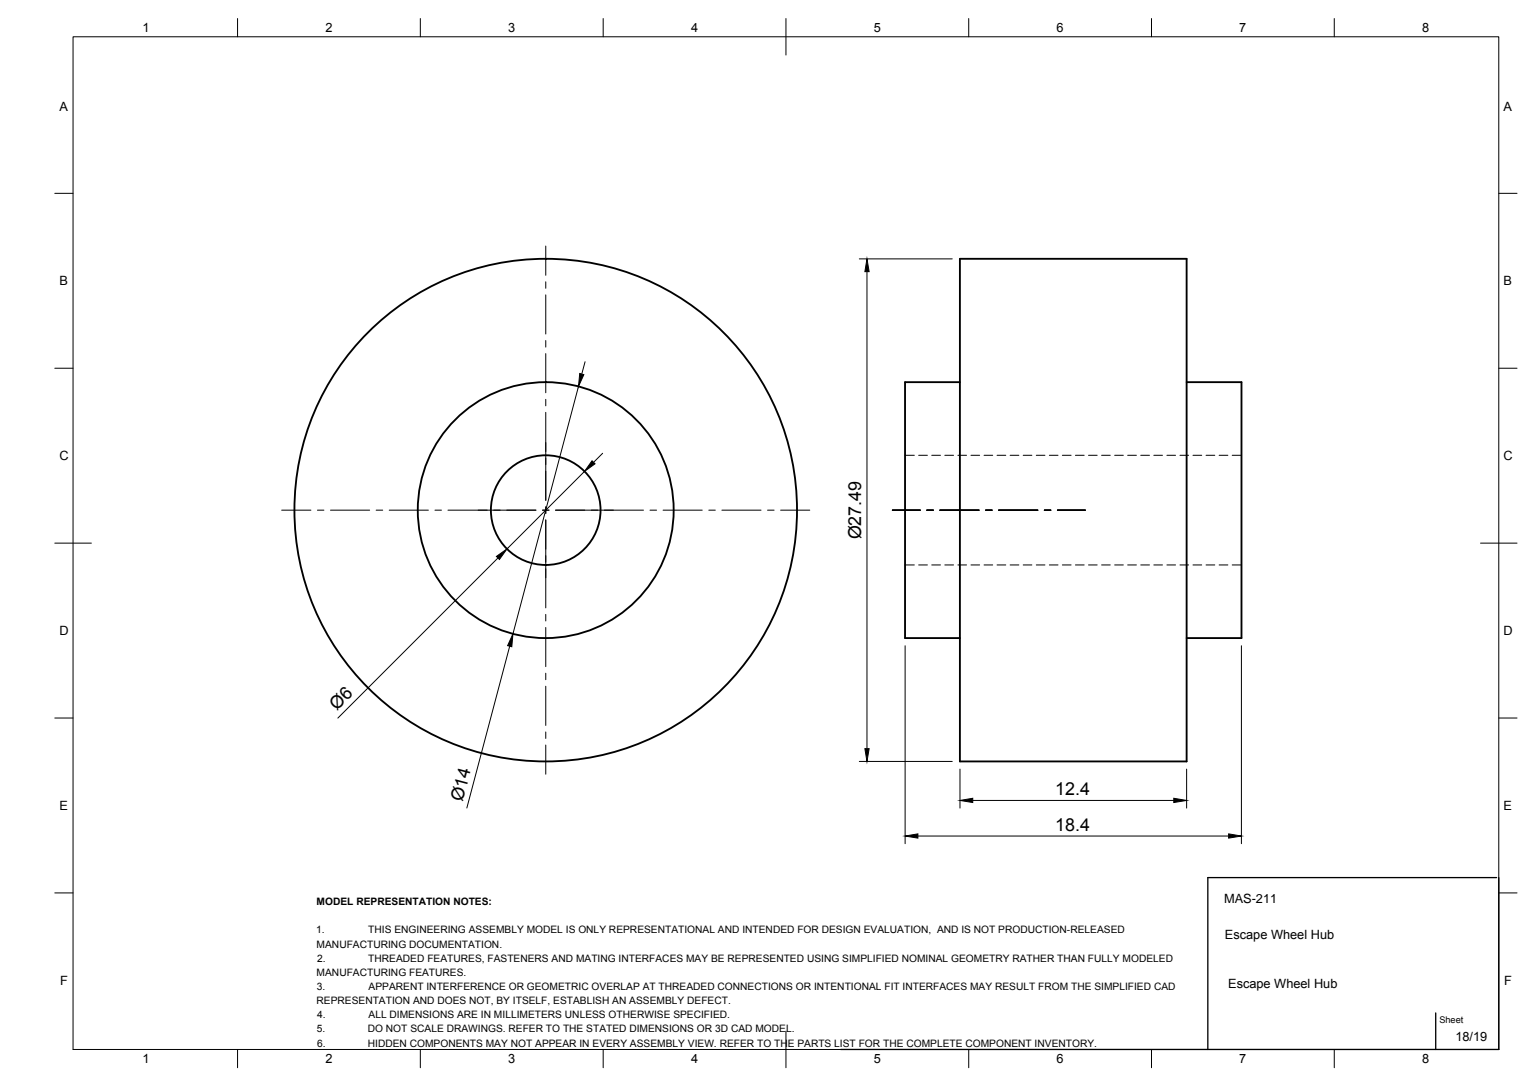
ISO-10303-21;
HEADER;
FILE_DESCRIPTION(
 (''),
 '2;1');
FILE_NAME ( 'Escape Wheel Hub.step', '2026-10-05T20:07:59+06:00', ( '' ), ( '' ), 'STEP AP214', 'Unspecified', '' );
FILE_SCHEMA (('AUTOMOTIVE_DESIGN { 1 0 10303 214 3 1 1 }'));
ENDSEC;
DATA;
#10=MECHANICAL_DESIGN_GEOMETRIC_PRESENTATION_REPRESENTATION('',(#336),#196741);
#336=STYLED_ITEM('',(#196765),#355) ;
#355=MANIFOLD_SOLID_BREP('Escape Wheel Hub',#8732) ;
#416=PLANE('',#9088) ;
#417=PLANE('',#9091) ;
#418=PLANE('',#9096) ;
#419=PLANE('',#9098) ;
#594=FACE_BOUND('',#1612,.T.) ;
#595=FACE_BOUND('',#1614,.T.) ;
#596=FACE_BOUND('',#1617,.T.) ;
#597=FACE_BOUND('',#1619,.T.) ;
#737=CIRCLE('',#9086,7.) ;
#738=CIRCLE('',#9087,7.) ;
#739=CIRCLE('',#9089,7.) ;
#740=CIRCLE('',#9090,3.00000000000006) ;
#741=CIRCLE('',#9092,3.00000000000006) ;
#742=CIRCLE('',#9094,13.7469842874597) ;
#743=CIRCLE('',#9095,13.7469842874597) ;
#744=CIRCLE('',#9097,7.) ;
#1097=FACE_OUTER_BOUND('',#1610,.T.) ;
#1098=FACE_OUTER_BOUND('',#1611,.T.) ;
#1099=FACE_OUTER_BOUND('',#1613,.T.) ;
#1100=FACE_OUTER_BOUND('',#1615,.T.) ;
#1101=FACE_OUTER_BOUND('',#1616,.T.) ;
#1102=FACE_OUTER_BOUND('',#1618,.T.) ;
#1103=FACE_OUTER_BOUND('',#1620,.T.) ;
#1104=FACE_OUTER_BOUND('',#1621,.T.) ;
#1610=EDGE_LOOP('',(#6758,#6759,#6760,#6761)) ;
#1611=EDGE_LOOP('',(#6762)) ;
#1612=EDGE_LOOP('',(#6763)) ;
#1613=EDGE_LOOP('',(#6764)) ;
#1614=EDGE_LOOP('',(#6765)) ;
#1615=EDGE_LOOP('',(#6766,#6767,#6768,#6769)) ;
#1616=EDGE_LOOP('',(#6770)) ;
#1617=EDGE_LOOP('',(#6771)) ;
#1618=EDGE_LOOP('',(#6772)) ;
#1619=EDGE_LOOP('',(#6773)) ;
#1620=EDGE_LOOP('',(#6774,#6775,#6776,#6777)) ;
#1621=EDGE_LOOP('',(#6778,#6779,#6780,#6781)) ;
#2079=LINE('',#194829,#2782) ;
#2080=LINE('',#194843,#2783) ;
#2081=LINE('',#194850,#2784) ;
#2082=LINE('',#194852,#2785) ;
#2782=VECTOR('',#10353,7.00000000000021) ;
#2783=VECTOR('',#10370,13.7469842874597) ;
#2784=VECTOR('',#10381,7.00000000000021) ;
#2785=VECTOR('',#10384,3.00000000000005) ;
#3838=VERTEX_POINT('',#194826) ;
#3839=VERTEX_POINT('',#194828) ;
#3840=VERTEX_POINT('',#194832) ;
#3841=VERTEX_POINT('',#194834) ;
#3842=VERTEX_POINT('',#194837) ;
#3843=VERTEX_POINT('',#194840) ;
#3844=VERTEX_POINT('',#194842) ;
#3845=VERTEX_POINT('',#194846) ;
#4887=EDGE_CURVE('',#3838,#3838,#737,.T.) ;
#4888=EDGE_CURVE('',#3838,#3839,#2079,.T.) ;
#4889=EDGE_CURVE('',#3839,#3839,#738,.T.) ;
#4890=EDGE_CURVE('',#3840,#3840,#739,.T.) ;
#4891=EDGE_CURVE('',#3841,#3841,#740,.T.) ;
#4892=EDGE_CURVE('',#3842,#3842,#741,.T.) ;
#4893=EDGE_CURVE('',#3843,#3843,#742,.T.) ;
#4894=EDGE_CURVE('',#3843,#3844,#2080,.T.) ;
#4895=EDGE_CURVE('',#3844,#3844,#743,.T.) ;
#4896=EDGE_CURVE('',#3845,#3845,#744,.T.) ;
#4897=EDGE_CURVE('',#3840,#3845,#2081,.T.) ;
#4898=EDGE_CURVE('',#3842,#3841,#2082,.T.) ;
#6758=ORIENTED_EDGE('',*,*,#4887,.T.) ;
#6759=ORIENTED_EDGE('',*,*,#4888,.T.) ;
#6760=ORIENTED_EDGE('',*,*,#4889,.F.) ;
#6761=ORIENTED_EDGE('',*,*,#4888,.F.) ;
#6762=ORIENTED_EDGE('',*,*,#4890,.F.) ;
#6763=ORIENTED_EDGE('',*,*,#4891,.F.) ;
#6764=ORIENTED_EDGE('',*,*,#4889,.T.) ;
#6765=ORIENTED_EDGE('',*,*,#4892,.T.) ;
#6766=ORIENTED_EDGE('',*,*,#4893,.T.) ;
#6767=ORIENTED_EDGE('',*,*,#4894,.T.) ;
#6768=ORIENTED_EDGE('',*,*,#4895,.F.) ;
#6769=ORIENTED_EDGE('',*,*,#4894,.F.) ;
#6770=ORIENTED_EDGE('',*,*,#4893,.F.) ;
#6771=ORIENTED_EDGE('',*,*,#4896,.T.) ;
#6772=ORIENTED_EDGE('',*,*,#4895,.T.) ;
#6773=ORIENTED_EDGE('',*,*,#4887,.F.) ;
#6774=ORIENTED_EDGE('',*,*,#4890,.T.) ;
#6775=ORIENTED_EDGE('',*,*,#4897,.T.) ;
#6776=ORIENTED_EDGE('',*,*,#4896,.F.) ;
#6777=ORIENTED_EDGE('',*,*,#4897,.F.) ;
#6778=ORIENTED_EDGE('',*,*,#4892,.F.) ;
#6779=ORIENTED_EDGE('',*,*,#4898,.T.) ;
#6780=ORIENTED_EDGE('',*,*,#4891,.T.) ;
#6781=ORIENTED_EDGE('',*,*,#4898,.F.) ;
#8205=CYLINDRICAL_SURFACE('',#9085,7.00000000000021) ;
#8206=CYLINDRICAL_SURFACE('',#9093,13.7469842874597) ;
#8207=CYLINDRICAL_SURFACE('',#9099,7.00000000000021) ;
#8208=CYLINDRICAL_SURFACE('',#9100,3.00000000000005) ;
#8480=ADVANCED_FACE('',(#1097),#8205,.T.) ;
#8481=ADVANCED_FACE('',(#1098,#594),#416,.T.) ;
#8482=ADVANCED_FACE('',(#1099,#595),#417,.T.) ;
#8483=ADVANCED_FACE('',(#1100),#8206,.T.) ;
#8484=ADVANCED_FACE('',(#1101,#596),#418,.T.) ;
#8485=ADVANCED_FACE('',(#1102,#597),#419,.T.) ;
#8486=ADVANCED_FACE('',(#1103),#8207,.T.) ;
#8487=ADVANCED_FACE('',(#1104),#8208,.F.) ;
#8732=CLOSED_SHELL('',(#8480,#8481,#8482,#8483,#8484,#8485,#8486,#8487)) ;
#9085=AXIS2_PLACEMENT_3D('',#194825,#10349,#10350) ;
#9086=AXIS2_PLACEMENT_3D('',#194827,#10351,#10352) ;
#9087=AXIS2_PLACEMENT_3D('',#194830,#10354,#10355) ;
#9088=AXIS2_PLACEMENT_3D('',#194831,#10356,#10357) ;
#9089=AXIS2_PLACEMENT_3D('',#194833,#10358,#10359) ;
#9090=AXIS2_PLACEMENT_3D('',#194835,#10360,#10361) ;
#9091=AXIS2_PLACEMENT_3D('',#194836,#10362,#10363) ;
#9092=AXIS2_PLACEMENT_3D('',#194838,#10364,#10365) ;
#9093=AXIS2_PLACEMENT_3D('',#194839,#10366,#10367) ;
#9094=AXIS2_PLACEMENT_3D('',#194841,#10368,#10369) ;
#9095=AXIS2_PLACEMENT_3D('',#194844,#10371,#10372) ;
#9096=AXIS2_PLACEMENT_3D('',#194845,#10373,#10374) ;
#9097=AXIS2_PLACEMENT_3D('',#194847,#10375,#10376) ;
#9098=AXIS2_PLACEMENT_3D('',#194848,#10377,#10378) ;
#9099=AXIS2_PLACEMENT_3D('',#194849,#10379,#10380) ;
#9100=AXIS2_PLACEMENT_3D('',#194851,#10382,#10383) ;
#10349=DIRECTION('center_axis',(0.,1.,0.)) ;
#10350=DIRECTION('ref_axis',(-0.623533159707219,0.,-0.78179690377075)) ;
#10351=DIRECTION('center_axis',(1.79188741038833E-16,-1.,-1.92949962064913E-16)) ;
#10352=DIRECTION('ref_axis',(0.961756409181177,1.58603289232165E-16,0.273906205477219)) ;
#10353=DIRECTION('',(0.,-1.,0.)) ;
#10354=DIRECTION('center_axis',(-2.4680833998183E-16,-1.,1.47919563675122E-16)) ;
#10355=DIRECTION('ref_axis',(0.961756409181177,-1.58603289232165E-16,0.273906205477219)) ;
#10356=DIRECTION('center_axis',(0.,1.,0.)) ;
#10357=DIRECTION('ref_axis',(0.,0.,1.)) ;
#10358=DIRECTION('center_axis',(0.,-1.,0.)) ;
#10359=DIRECTION('ref_axis',(0.961756409181177,0.,0.273906205477219)) ;
#10360=DIRECTION('center_axis',(4.42840651093008E-17,1.,1.84317809555473E-16)) ;
#10361=DIRECTION('ref_axis',(-0.0741867580339816,0.,0.997244365706023)) ;
#10362=DIRECTION('center_axis',(0.,-1.,0.)) ;
#10363=DIRECTION('ref_axis',(0.,0.,-1.)) ;
#10364=DIRECTION('center_axis',(-4.42840651093008E-17,1.,-1.84317809555473E-16)) ;
#10365=DIRECTION('ref_axis',(-0.0741867580339816,0.,0.997244365706023)) ;
#10366=DIRECTION('center_axis',(0.,1.,0.)) ;
#10367=DIRECTION('ref_axis',(0.69769452851967,0.,-0.716395383062813)) ;
#10368=DIRECTION('center_axis',(-1.84442498271352E-17,-1.,3.70289586508121E-17)) ;
#10369=DIRECTION('ref_axis',(-0.15149846795078,0.,0.988457492363008)) ;
#10370=DIRECTION('',(0.,-1.,0.)) ;
#10371=DIRECTION('center_axis',(-1.08888592718918E-16,-1.,-7.82420061571595E-17)) ;
#10372=DIRECTION('ref_axis',(-0.15149846795078,-8.07612056149597E-17,0.988457492363008)) ;
#10373=DIRECTION('center_axis',(0.,1.,0.)) ;
#10374=DIRECTION('ref_axis',(0.,0.,1.)) ;
#10375=DIRECTION('center_axis',(0.,-1.,0.)) ;
#10376=DIRECTION('ref_axis',(0.961756409181177,0.,0.273906205477219)) ;
#10377=DIRECTION('center_axis',(0.,-1.,0.)) ;
#10378=DIRECTION('ref_axis',(0.,0.,-1.)) ;
#10379=DIRECTION('center_axis',(0.,1.,0.)) ;
#10380=DIRECTION('ref_axis',(-0.623533159707219,0.,-0.78179690377075)) ;
#10381=DIRECTION('',(0.,-1.,0.)) ;
#10382=DIRECTION('center_axis',(0.,-1.,0.)) ;
#10383=DIRECTION('ref_axis',(0.519132143162,0.,0.854693990815443)) ;
#10384=DIRECTION('',(0.,1.,0.)) ;
#194825=CARTESIAN_POINT('Origin',(2.26485497023532E-13,9.2000000000496,
130.056003483261)) ;
#194826=CARTESIAN_POINT('',(4.36473211795044,-6.19999999995041,135.528581809656)) ;
#194827=CARTESIAN_POINT('Origin',(5.55111512312578E-16,-6.19999999995041,
130.056003483261)) ;
#194828=CARTESIAN_POINT('',(4.36473211795044,-9.1999999999504,135.528581809656)) ;
#194829=CARTESIAN_POINT('',(4.36473211795089,9.2000000000496,135.528581809656)) ;
#194830=CARTESIAN_POINT('Origin',(5.55111512312578E-16,-9.1999999999504,
130.056003483261)) ;
#194831=CARTESIAN_POINT('Origin',(4.36473211795044,9.2000000000496,135.528581809656)) ;
#194832=CARTESIAN_POINT('',(4.36473211795044,9.2000000000496,135.528581809656)) ;
#194833=CARTESIAN_POINT('Origin',(5.55111512312578E-16,9.2000000000496,
130.056003483261)) ;
#194834=CARTESIAN_POINT('',(-1.55739642948599,9.2000000000496,127.491921510814)) ;
#194835=CARTESIAN_POINT('Origin',(9.54791801177635E-14,9.2000000000496,
130.056003483261)) ;
#194836=CARTESIAN_POINT('Origin',(4.36473211795044,-9.1999999999504,135.528581809656)) ;
#194837=CARTESIAN_POINT('',(-1.55739642948599,-9.19999999995041,127.491921510814)) ;
#194838=CARTESIAN_POINT('Origin',(9.54791801177635E-14,-9.19999999995041,
130.056003483261)) ;
#194839=CARTESIAN_POINT('Origin',(1.99840144432528E-14,6.2000000000496,
130.056003483261)) ;
#194840=CARTESIAN_POINT('',(-9.59119572100644,6.2000000000496,139.904279557834)) ;
#194841=CARTESIAN_POINT('Origin',(1.34336985979644E-13,6.2000000000496,
130.056003483261)) ;
#194842=CARTESIAN_POINT('',(-9.59119572100644,-6.19999999995041,139.904279557834)) ;
#194843=CARTESIAN_POINT('',(-9.59119572100651,6.2000000000496,139.904279557834)) ;
#194844=CARTESIAN_POINT('Origin',(1.34336985979644E-13,-6.19999999995041,
130.056003483261)) ;
#194845=CARTESIAN_POINT('Origin',(-9.59119572100644,6.2000000000496,139.904279557834)) ;
#194846=CARTESIAN_POINT('',(4.36473211795044,6.2000000000496,135.528581809656)) ;
#194847=CARTESIAN_POINT('Origin',(5.55111512312578E-16,6.2000000000496,
130.056003483261)) ;
#194848=CARTESIAN_POINT('Origin',(-9.59119572100644,-6.19999999995041,139.904279557834)) ;
#194849=CARTESIAN_POINT('Origin',(2.26485497023532E-13,9.2000000000496,
130.056003483261)) ;
#194850=CARTESIAN_POINT('',(4.36473211795089,9.2000000000496,135.528581809656)) ;
#194851=CARTESIAN_POINT('Origin',(3.60822483003176E-14,4.9595882956055E-11,
130.056003483261)) ;
#194852=CARTESIAN_POINT('',(-1.55739642948599,4.9595882956055E-11,127.491921510814)) ;
#196737=UNCERTAINTY_MEASURE_WITH_UNIT(LENGTH_MEASURE(0.01),#196742,
'DISTANCE_ACCURACY_VALUE',
'Maximum model space distance between geometric entities at asserted c
onnectivities') ;
#196738=UNCERTAINTY_MEASURE_WITH_UNIT(LENGTH_MEASURE(0.01),#196742,
'DISTANCE_ACCURACY_VALUE',
'Maximum model space distance between geometric entities at asserted c
onnectivities') ;
#196740=(
GEOMETRIC_REPRESENTATION_CONTEXT(3)
GLOBAL_UNCERTAINTY_ASSIGNED_CONTEXT((#196737))
GLOBAL_UNIT_ASSIGNED_CONTEXT((#196742,#196744,#196745))
REPRESENTATION_CONTEXT('','3D')
) ;
#196741=(
GEOMETRIC_REPRESENTATION_CONTEXT(3)
GLOBAL_UNCERTAINTY_ASSIGNED_CONTEXT((#196738))
GLOBAL_UNIT_ASSIGNED_CONTEXT((#196742,#196744,#196745))
REPRESENTATION_CONTEXT('','3D')
) ;
#196742=(
LENGTH_UNIT()
NAMED_UNIT(*)
SI_UNIT(.MILLI.,.METRE.)
) ;
#196744=(
NAMED_UNIT(*)
PLANE_ANGLE_UNIT()
SI_UNIT($,.RADIAN.)
) ;
#196745=(
NAMED_UNIT(*)
SI_UNIT($,.STERADIAN.)
SOLID_ANGLE_UNIT()
) ;
#196753=PRODUCT_DEFINITION_CONTEXT('part definition',#196761,'design') ;
#196761=APPLICATION_CONTEXT(
'Core Data for Automotive Mechanical Design Process') ;
#196762=PRODUCT_CONTEXT('part definition',#196761,'mechanical') ;
#196765=PRESENTATION_STYLE_ASSIGNMENT((#196767)) ;
#196767=SURFACE_STYLE_USAGE(.BOTH.,#196769) ;
#196769=SURFACE_SIDE_STYLE('',(#196771)) ;
#196771=SURFACE_STYLE_FILL_AREA(#196773) ;
#196773=FILL_AREA_STYLE('Steel - Satin',(#196775)) ;
#196775=FILL_AREA_STYLE_COLOUR('Steel - Satin',#196777) ;
#196777=COLOUR_RGB('Steel - Satin', 0.09019608, 0.27058824, 0.51372549) ;
#197187=CARTESIAN_POINT ( '', ( 0.0, 0.0, 0.0 ) ) ;
#197188=DIRECTION ( '', ( 0.0, 0.0, 1.0 ) ) ;
#197189=DIRECTION ( '', ( 1.0, 0.0, 0.0 ) ) ;
#197190=AXIS2_PLACEMENT_3D ( '', #197187, #197188, #197189 ) ;
#197191=ADVANCED_BREP_SHAPE_REPRESENTATION ( 'Escape Wheel Hub', ( #355, #197190, #197201, #197459 ), #196740 ) ;
#197192=PRODUCT( 'Escape Wheel Hub', 'Escape Wheel Hub', '', ( #196762 ) ) ;
#197193=PRODUCT_DEFINITION_FORMATION ( '', '', #197192 ) ;
#197194=PRODUCT_DEFINITION( 'Escape Wheel Hub', 'Escape Wheel Hub', #197193, #196753 ) ;
#197195=PRODUCT_DEFINITION_SHAPE ( '', '', #197194 ) ;
#197196=SHAPE_DEFINITION_REPRESENTATION ( #197195, #197191 ) ;
#197198=CARTESIAN_POINT ( '', ( 0.0, 0.0, 0.0 ) ) ;
#197199=DIRECTION ( '', ( 0.0, 0.0, 1.0 ) ) ;
#197200=DIRECTION ( '', ( 1.0, 0.0, 0.0 ) ) ;
#197201=AXIS2_PLACEMENT_3D ( '', #197198, #197199, #197200 ) ;
#197456=CARTESIAN_POINT ( '', ( 0.0, 0.0, 0.0 ) ) ;
#197457=DIRECTION ( '', ( 0.0, 0.0, 1.0 ) ) ;
#197458=DIRECTION ( '', ( 1.0, 0.0, 0.0 ) ) ;
#197459=AXIS2_PLACEMENT_3D ( '', #197456, #197457, #197458 ) ;
ENDSEC;
END-ISO-10303-21;
